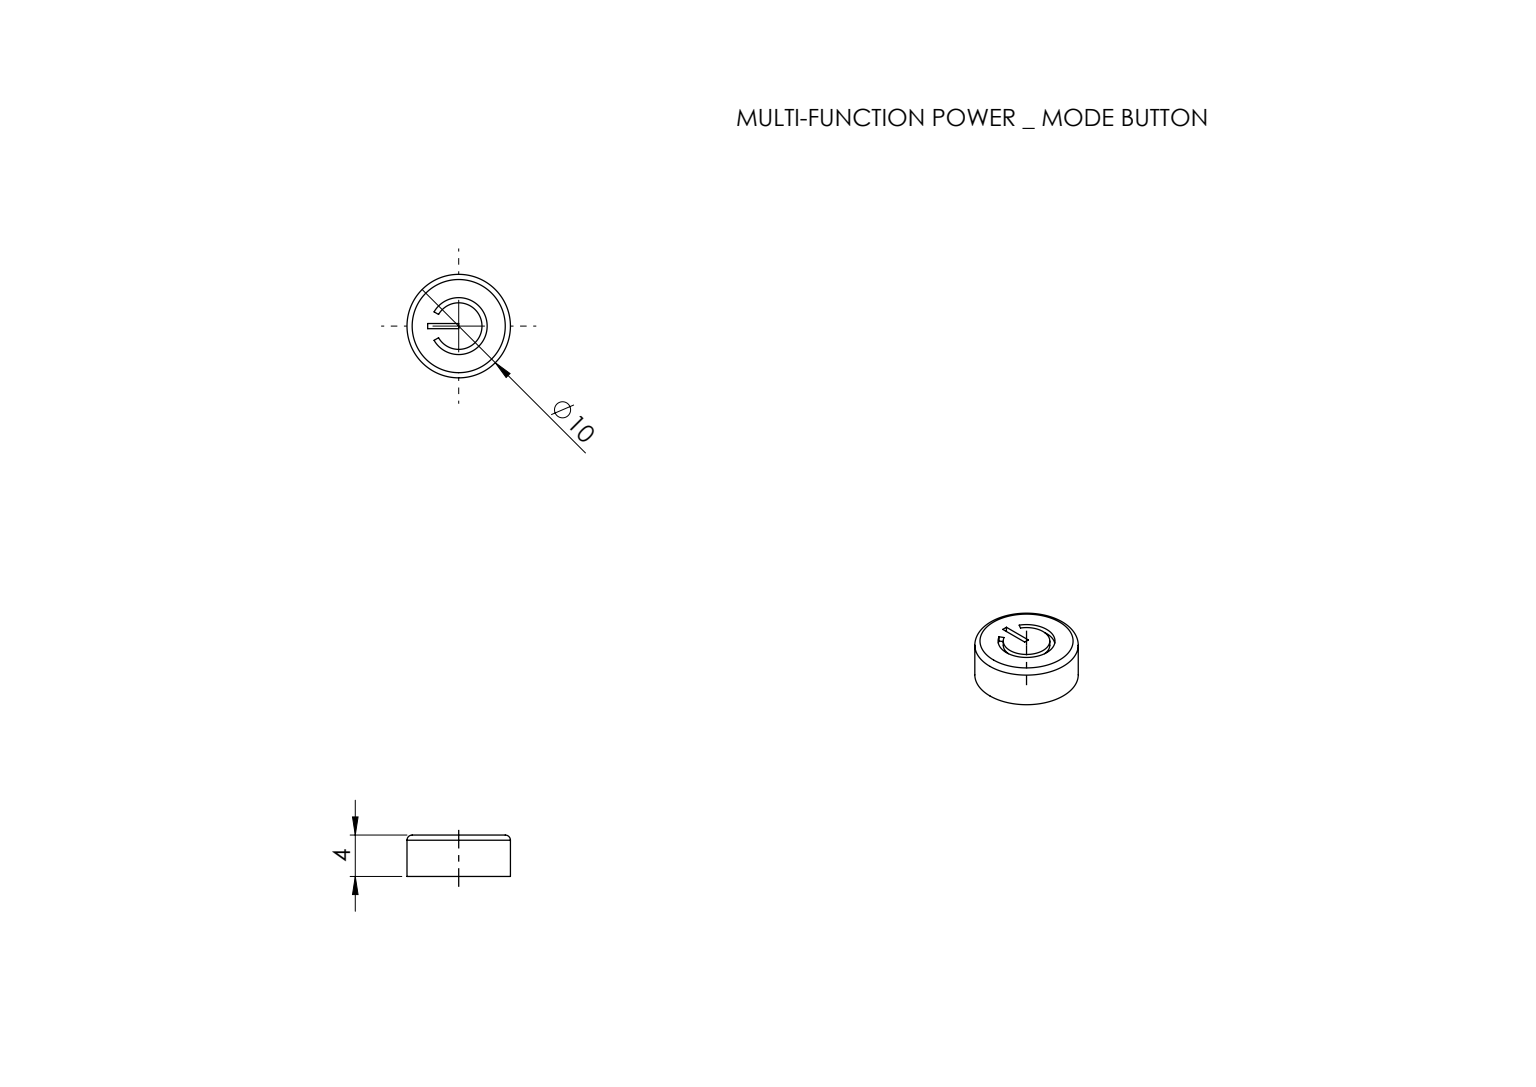
ISO-10303-21;
HEADER;
FILE_DESCRIPTION (('STEP AP214'),
    '1' );
FILE_NAME ('Multi-Function Power _ Mode Button.step',
    '2026-10-02T09:26:43',
    ( '' ),
    ( '' ),
    'SwSTEP 2.0',
    'SolidWorks 2026',
    '' );
FILE_SCHEMA (( 'AUTOMOTIVE_DESIGN' ));
ENDSEC;

DATA;
#385=ORIENTED_EDGE ( 'NONE', *, *, #77434, .T. ) ;
#488=DIRECTION ( 'NONE',  ( 1.000000000000000000, 0.000000000000000000, 0.000000000000000000 ) ) ;
#790=DIRECTION ( 'NONE',  ( -0.000000000000000000, -1.000000000000000000, -0.000000000000000000 ) ) ;
#881=DIRECTION ( 'NONE',  ( -0.000000000000000000, -1.000000000000000000, -0.000000000000000000 ) ) ;
#1377=EDGE_CURVE ( 'NONE', #21459, #55389, #67444, .T. ) ;
#1508=( NAMED_UNIT ( * ) SI_UNIT ( $, .STERADIAN. ) SOLID_ANGLE_UNIT ( ) );
#1978=( LENGTH_UNIT ( ) NAMED_UNIT ( * ) SI_UNIT ( .MILLI., .METRE. ) );
#2148=VERTEX_POINT ( 'NONE', #84417 ) ;
#2193=DIRECTION ( 'NONE',  ( -0.000000000000000000, -1.000000000000000000, -0.000000000000000000 ) ) ;
#2267=VERTEX_POINT ( 'NONE', #109201 ) ;
#2382=DIRECTION ( 'NONE',  ( 0.000000000000000000, 0.000000000000000000, 1.000000000000000000 ) ) ;
#2384=UNCERTAINTY_MEASURE_WITH_UNIT (LENGTH_MEASURE( 1.000000000000000082E-05 ), #1978, 'distance_accuracy_value', 'NONE');
#2834=APPLICATION_CONTEXT ( 'automotive_design' ) ;
#3149=ORIENTED_EDGE ( 'NONE', *, *, #1377, .F. ) ;
#3203=DIRECTION ( 'NONE',  ( -1.000000000000000000, 0.000000000000000000, 1.224646799147352221E-16 ) ) ;
#3290=DIRECTION ( 'NONE',  ( -0.000000000000000000, -1.000000000000000000, -0.000000000000000000 ) ) ;
#3313=ORIENTED_EDGE ( 'NONE', *, *, #12967, .T. ) ;
#3340=ORIENTED_EDGE ( 'NONE', *, *, #86447, .T. ) ;
#3667=CARTESIAN_POINT ( 'NONE',  ( 105.6184301395928031, 8.500000000000000000, -1.375000000000000888 ) ) ;
#3718=ORIENTED_EDGE ( 'NONE', *, *, #81749, .T. ) ;
#3750=CARTESIAN_POINT ( 'NONE',  ( 106.0514428414850272, 8.500000000000000000, -1.125000000000000222 ) ) ;
#3830=DIRECTION ( 'NONE',  ( -1.224646799147352221E-16, 0.000000000000000000, -1.000000000000000000 ) ) ;
#3880=CIRCLE ( 'NONE', #6023, 0.5000000000000004441 ) ;
#4515=LINE ( 'NONE', #115118, #126781 ) ;
#4690=DIRECTION ( 'NONE',  ( -0.000000000000000000, 1.000000000000000000, -0.000000000000000000 ) ) ;
#4889=EDGE_CURVE ( 'NONE', #106872, #121536, #118797, .T. ) ;
#4891=AXIS2_PLACEMENT_3D ( 'NONE', #71967, #92220, #82437 ) ;
#5329=CARTESIAN_POINT ( 'NONE',  ( 108.0000000000000142, 8.500000000000000000, 0.000000000000000000 ) ) ;
#5405=CARTESIAN_POINT ( 'NONE',  ( 105.0000000000000142, 8.500000000000000000, -0.2499999999999996392 ) ) ;
#5772=CARTESIAN_POINT ( 'NONE',  ( 108.0000000000000142, 5.000000000000000000, 0.000000000000000000 ) ) ;
#5797=EDGE_LOOP ( 'NONE', ( #22080, #113484 ) ) ;
#5964=DIRECTION ( 'NONE',  ( -0.000000000000000000, -1.000000000000000000, -0.000000000000000000 ) ) ;
#5971=( GEOMETRIC_REPRESENTATION_CONTEXT ( 3 ) GLOBAL_UNCERTAINTY_ASSIGNED_CONTEXT ( ( #2384 ) ) GLOBAL_UNIT_ASSIGNED_CONTEXT ( ( #1978, #22299, #60295 ) ) REPRESENTATION_CONTEXT ( 'NONE', 'WORKASPACE' ) );
#5975=FACE_OUTER_BOUND ( 'NONE', #11208, .T. ) ;
#6023=AXIS2_PLACEMENT_3D ( 'NONE', #88627, #38920, #50635 ) ;
#6047=UNCERTAINTY_MEASURE_WITH_UNIT (LENGTH_MEASURE( 1.000000000000000082E-05 ), #11976, 'distance_accuracy_value', 'NONE');
#6325=ORIENTED_EDGE ( 'NONE', *, *, #106005, .T. ) ;
#8150=EDGE_CURVE ( 'NONE', #2148, #54782, #127046, .T. ) ;
#8522=EDGE_CURVE ( 'NONE', #106872, #41830, #78934, .T. ) ;
#8952=ORIENTED_EDGE ( 'NONE', *, *, #89643, .T. ) ;
#8954=AXIS2_PLACEMENT_3D ( 'NONE', #36524, #76432, #77074 ) ;
#9891=ORIENTED_EDGE ( 'NONE', *, *, #89462, .T. ) ;
#10025=VERTEX_POINT ( 'NONE', #92625 ) ;
#10069=DIRECTION ( 'NONE',  ( 0.000000000000000000, -0.000000000000000000, 1.000000000000000000 ) ) ;
#10097=CARTESIAN_POINT ( 'NONE',  ( 108.0000000000000142, 8.500000000000000000, 0.000000000000000000 ) ) ;
#10308=VERTEX_POINT ( 'NONE', #14043 ) ;
#10568=EDGE_CURVE ( 'NONE', #72837, #121539, #100366, .T. ) ;
#10644=CARTESIAN_POINT ( 'NONE',  ( 0.000000000000000000, 0.000000000000000000, 0.000000000000000000 ) ) ;
#10960=ORIENTED_EDGE ( 'NONE', *, *, #81749, .F. ) ;
#11208=EDGE_LOOP ( 'NONE', ( #44989, #6325, #121739, #15666 ) ) ;
#11396=ORIENTED_EDGE ( 'NONE', *, *, #79481, .F. ) ;
#11481=CARTESIAN_POINT ( 'NONE',  ( 108.0000000000000142, 9.000000000000001776, 4.500000000000003553 ) ) ;
#11637=DIRECTION ( 'NONE',  ( 0.000000000000000000, 1.000000000000000000, 0.000000000000000000 ) ) ;
#11693=CYLINDRICAL_SURFACE ( 'NONE', #74639, 2.749999999999997335 ) ;
#11728=ADVANCED_FACE ( 'NONE', ( #29081, #57229, #39562 ), #19222, .T. ) ;
#11976=( LENGTH_UNIT ( ) NAMED_UNIT ( * ) SI_UNIT ( .MILLI., .METRE. ) );
#12204=CARTESIAN_POINT ( 'NONE',  ( 108.0000000000000142, 9.000000000000001776, 5.000000000000004441 ) ) ;
#12216=CARTESIAN_POINT ( 'NONE',  ( 108.0000000000000142, 5.000000000000000000, 0.000000000000000000 ) ) ;
#12407=CARTESIAN_POINT ( 'NONE',  ( 108.0000000000000142, 8.500000000000000000, 2.249999999999996891 ) ) ;
#12614=PRESENTATION_STYLE_ASSIGNMENT (( #61086 ) ) ;
#12967=EDGE_CURVE ( 'NONE', #112645, #70298, #25079, .T. ) ;
#12984=DIRECTION ( 'NONE',  ( 0.000000000000000000, 0.000000000000000000, 1.000000000000000000 ) ) ;
#13074=( NAMED_UNIT ( * ) PLANE_ANGLE_UNIT ( ) SI_UNIT ( $, .RADIAN. ) );
#13182=DIRECTION ( 'NONE',  ( 0.000000000000000000, 0.000000000000000000, 1.000000000000000000 ) ) ;
#13266=ORIENTED_EDGE ( 'NONE', *, *, #55211, .T. ) ;
#13423=ORIENTED_EDGE ( 'NONE', *, *, #70420, .F. ) ;
#13659=DIRECTION ( 'NONE',  ( 0.4999999999999992228, 0.000000000000000000, -0.8660254037844391517 ) ) ;
#13797=DIRECTION ( 'NONE',  ( -0.000000000000000000, 1.000000000000000000, -0.000000000000000000 ) ) ;
#13876=DIRECTION ( 'NONE',  ( -0.000000000000000000, -1.000000000000000000, -0.000000000000000000 ) ) ;
#14043=CARTESIAN_POINT ( 'NONE',  ( 106.0514428414850272, 9.000000000000001776, 1.124999999999998002 ) ) ;
#15131=DIRECTION ( 'NONE',  ( 1.000000000000000000, 0.000000000000000000, -1.776356839400246520E-15 ) ) ;
#15253=ORIENTED_EDGE ( 'NONE', *, *, #113422, .F. ) ;
#15666=ORIENTED_EDGE ( 'NONE', *, *, #93447, .F. ) ;
#16016=CARTESIAN_POINT ( 'NONE',  ( 105.6184301395928031, 9.000000000000001776, 1.375000000000001110 ) ) ;
#16189=APPLICATION_CONTEXT ( 'automotive_design' ) ;
#16276=ADVANCED_FACE ( 'NONE', ( #21523 ), #11693, .F. ) ;
#16605=EDGE_CURVE ( 'NONE', #74101, #10308, #73370, .T. ) ;
#16684=VECTOR ( 'NONE', #13797, 1000.000000000000000 ) ;
#17289=DIRECTION ( 'NONE',  ( 0.8660254037844390407, 0.000000000000000000, -0.4999999999999991673 ) ) ;
#17307=CIRCLE ( 'NONE', #46578, 5.000000000000004441 ) ;
#17535=FACE_OUTER_BOUND ( 'NONE', #5797, .T. ) ;
#17646=AXIS2_PLACEMENT_3D ( 'NONE', #126359, #117804, #56948 ) ;
#17782=EDGE_LOOP ( 'NONE', ( #128177, #26734, #108737, #88245 ) ) ;
#17911=DIRECTION ( 'NONE',  ( 1.000000000000000000, 0.000000000000000000, 8.881784197001235560E-16 ) ) ;
#18235=LINE ( 'NONE', #70561, #41090 ) ;
#18489=ADVANCED_FACE ( 'NONE', ( #17535 ), #75813, .F. ) ;
#18780=CARTESIAN_POINT ( 'NONE',  ( 105.0000000000000142, 9.000000000000001776, 0.2500000000000003886 ) ) ;
#19087=CARTESIAN_POINT ( 'NONE',  ( 108.0000000000000142, 8.500000000000000000, 0.000000000000000000 ) ) ;
#19205=DIRECTION ( 'NONE',  ( -1.000000000000000000, 0.000000000000000000, 1.224646799147352221E-16 ) ) ;
#19222=PLANE ( 'NONE',  #63419 ) ;
#19401=AXIS2_PLACEMENT_3D ( 'NONE', #5772, #126869, #26096 ) ;
#19403=ORIENTED_EDGE ( 'NONE', *, *, #117219, .T. ) ;
#19505=EDGE_LOOP ( 'NONE', ( #103192, #97868, #89992, #40928 ) ) ;
#19520=DIRECTION ( 'NONE',  ( 0.000000000000000000, 0.000000000000000000, 1.000000000000000000 ) ) ;
#19573=AXIS2_PLACEMENT_3D ( 'NONE', #91743, #83223, #102836 ) ;
#19603=CARTESIAN_POINT ( 'NONE',  ( 108.0000000000000142, 9.000000000000001776, -5.000000000000004441 ) ) ;
#19610=DIRECTION ( 'NONE',  ( -0.000000000000000000, 1.000000000000000000, -0.000000000000000000 ) ) ;
#20007=DIRECTION ( 'NONE',  ( -1.000000000000000000, 0.000000000000000000, 1.224646799147352221E-16 ) ) ;
#20093=LINE ( 'NONE', #89473, #27972 ) ;
#20109=DIRECTION ( 'NONE',  ( -0.000000000000000000, -1.000000000000000000, -0.000000000000000000 ) ) ;
#21087=VECTOR ( 'NONE', #20109, 1000.000000000000000 ) ;
#21272=PRODUCT_DEFINITION_FORMATION_WITH_SPECIFIED_SOURCE ( 'ANY', '', #72268, .NOT_KNOWN. ) ;
#21349=DIRECTION ( 'NONE',  ( 1.000000000000000000, 0.000000000000000000, 8.881784197001235560E-16 ) ) ;
#21459=VERTEX_POINT ( 'NONE', #91482 ) ;
#21523=FACE_OUTER_BOUND ( 'NONE', #121290, .T. ) ;
#21874=VERTEX_POINT ( 'NONE', #11481 ) ;
#22080=ORIENTED_EDGE ( 'NONE', *, *, #114243, .F. ) ;
#22299=( NAMED_UNIT ( * ) PLANE_ANGLE_UNIT ( ) SI_UNIT ( $, .RADIAN. ) );
#22796=VECTOR ( 'NONE', #17289, 1000.000000000000227 ) ;
#22913=LINE ( 'NONE', #62831, #59996 ) ;
#23418=CIRCLE ( 'NONE', #48569, 2.750000000000002665 ) ;
#23447=DIRECTION ( 'NONE',  ( -0.000000000000000000, 1.000000000000000000, -0.000000000000000000 ) ) ;
#23521=CARTESIAN_POINT ( 'NONE',  ( 106.0514428414850272, 8.500000000000000000, 1.125000000000000444 ) ) ;
#23569=CARTESIAN_POINT ( 'NONE',  ( 108.0000000000000142, 9.000000000000001776, 0.000000000000000000 ) ) ;
#24135=DIRECTION ( 'NONE',  ( 0.000000000000000000, 0.000000000000000000, 1.000000000000000000 ) ) ;
#24517=CIRCLE ( 'NONE', #106077, 2.250000000000001776 ) ;
#24540=ORIENTED_EDGE ( 'NONE', *, *, #98030, .T. ) ;
#24891=CARTESIAN_POINT ( 'NONE',  ( 108.0000000000000142, 9.000000000000001776, -0.2500000000000000000 ) ) ;
#24976=EDGE_LOOP ( 'NONE', ( #85852, #95541, #46748, #54051, #3149, #85174, #50534, #49698 ) ) ;
#25079=LINE ( 'NONE', #114103, #116619 ) ;
#25272=DIRECTION ( 'NONE',  ( -0.000000000000000000, -1.000000000000000000, -0.000000000000000000 ) ) ;
#25381=ORIENTED_EDGE ( 'NONE', *, *, #48110, .T. ) ;
#25558=ORIENTED_EDGE ( 'NONE', *, *, #55661, .F. ) ;
#25818=ORIENTED_EDGE ( 'NONE', *, *, #48110, .F. ) ;
#25918=CARTESIAN_POINT ( 'NONE',  ( 108.0000000000000142, 8.500000000000000000, 0.000000000000000000 ) ) ;
#26066=CARTESIAN_POINT ( 'NONE',  ( 108.0000000000000142, 9.000000000000001776, -0.2500000000000000000 ) ) ;
#26096=DIRECTION ( 'NONE',  ( 0.000000000000000000, -0.000000000000000000, 1.000000000000000000 ) ) ;
#26734=ORIENTED_EDGE ( 'NONE', *, *, #117792, .F. ) ;
#26804=EDGE_CURVE ( 'NONE', #109687, #10308, #34412, .T. ) ;
#26823=ORIENTED_EDGE ( 'NONE', *, *, #33540, .F. ) ;
#27919=DIRECTION ( 'NONE',  ( 1.000000000000000000, 0.000000000000000000, 1.776356839400247112E-15 ) ) ;
#27972=VECTOR ( 'NONE', #61953, 1000.000000000000000 ) ;
#28111=ORIENTED_EDGE ( 'NONE', *, *, #83838, .T. ) ;
#28210=EDGE_LOOP ( 'NONE', ( #77891, #123182, #92206, #99342 ) ) ;
#29081=FACE_BOUND ( 'NONE', #88903, .T. ) ;
#29085=EDGE_CURVE ( 'NONE', #55389, #74101, #108331, .T. ) ;
#30179=SHAPE_REPRESENTATION_RELATIONSHIP ( 'NONE' , 'NONE' ,  #89551, #108597 ) ;
#30252=DIRECTION ( 'NONE',  ( 1.000000000000000000, 0.000000000000000000, 0.000000000000000000 ) ) ;
#30311=ORIENTED_EDGE ( 'NONE', *, *, #113227, .T. ) ;
#30359=LINE ( 'NONE', #101005, #116796 ) ;
#30746=CIRCLE ( 'NONE', #124816, 4.500000000000003553 ) ;
#30906=DIRECTION ( 'NONE',  ( -1.000000000000000000, 0.000000000000000000, 0.000000000000000000 ) ) ;
#31194=CARTESIAN_POINT ( 'NONE',  ( 108.0000000000000142, 9.000000000000001776, 0.000000000000000000 ) ) ;
#31397=FACE_OUTER_BOUND ( 'NONE', #28210, .T. ) ;
#31472=CARTESIAN_POINT ( 'NONE',  ( 108.0000000000000142, 9.000000000000001776, -0.2500000000000000000 ) ) ;
#31821=CARTESIAN_POINT ( 'NONE',  ( 105.0000000000000142, 8.500000000000000000, 0.2500000000000003886 ) ) ;
#32513=DIRECTION ( 'NONE',  ( -0.000000000000000000, 1.000000000000000000, -0.000000000000000000 ) ) ;
#33199=STYLED_ITEM ( 'NONE', ( #70731 ), #108597 ) ;
#33298=ORIENTED_EDGE ( 'NONE', *, *, #4889, .F. ) ;
#33482=AXIS2_PLACEMENT_3D ( 'NONE', #47716, #69261, #120319 ) ;
#33540=EDGE_CURVE ( 'NONE', #55389, #56667, #109269, .T. ) ;
#33800=DIRECTION ( 'NONE',  ( 0.000000000000000000, 1.000000000000000000, 0.000000000000000000 ) ) ;
#34131=ORIENTED_EDGE ( 'NONE', *, *, #114243, .T. ) ;
#34206=ORIENTED_EDGE ( 'NONE', *, *, #117219, .F. ) ;
#34412=CIRCLE ( 'NONE', #122223, 2.250000000000001776 ) ;
#34634=ORIENTED_EDGE ( 'NONE', *, *, #12967, .F. ) ;
#34781=ADVANCED_FACE ( 'NONE', ( #31397 ), #61505, .T. ) ;
#34787=ADVANCED_FACE ( 'NONE', ( #113814 ), #94164, .T. ) ;
#34828=DIRECTION ( 'NONE',  ( 1.000000000000000000, 0.000000000000000000, -8.881784197001232602E-16 ) ) ;
#34919=VECTOR ( 'NONE', #67830, 1000.000000000000227 ) ;
#35042=AXIS2_PLACEMENT_3D ( 'NONE', #10097, #110231, #48095 ) ;
#35244=CARTESIAN_POINT ( 'NONE',  ( 108.0000000000000142, 8.500000000000000000, 0.000000000000000000 ) ) ;
#35998=VECTOR ( 'NONE', #104719, 1000.000000000000000 ) ;
#36343=CARTESIAN_POINT ( 'NONE',  ( 105.0000000000000142, 8.500000000000000000, 0.2500000000000003886 ) ) ;
#36524=CARTESIAN_POINT ( 'NONE',  ( 108.0000000000000142, 8.500000000000000000, -0.2500000000000000000 ) ) ;
#37026=DIRECTION ( 'NONE',  ( -0.000000000000000000, 1.000000000000000000, -0.000000000000000000 ) ) ;
#37092=AXIS2_PLACEMENT_3D ( 'NONE', #49730, #83052, #12984 ) ;
#37163=PLANE ( 'NONE',  #8954 ) ;
#37321=AXIS2_PLACEMENT_3D ( 'NONE', #5329, #5964, #15131 ) ;
#37329=AXIS2_PLACEMENT_3D ( 'NONE', #73402, #102854, #13182 ) ;
#37832=ORIENTED_EDGE ( 'NONE', *, *, #102627, .F. ) ;
#38166=VECTOR ( 'NONE', #102869, 1000.000000000000000 ) ;
#38625=CARTESIAN_POINT ( 'NONE',  ( 108.0000000000000142, 9.000000000000001776, -2.749999999999997335 ) ) ;
#38888=DIRECTION ( 'NONE',  ( -0.000000000000000000, -1.000000000000000000, -0.000000000000000000 ) ) ;
#38920=DIRECTION ( 'NONE',  ( 1.000000000000000000, -0.000000000000000000, 1.224646799147353207E-16 ) ) ;
#39345=ORIENTED_EDGE ( 'NONE', *, *, #58572, .T. ) ;
#39562=FACE_OUTER_BOUND ( 'NONE', #40627, .T. ) ;
#39567=ORIENTED_EDGE ( 'NONE', *, *, #58572, .F. ) ;
#40182=CARTESIAN_POINT ( 'NONE',  ( 108.0000000000000142, 9.000000000000001776, 0.000000000000000000 ) ) ;
#40340=ORIENTED_EDGE ( 'NONE', *, *, #84111, .F. ) ;
#40627=EDGE_LOOP ( 'NONE', ( #65864, #59906 ) ) ;
#40750=CARTESIAN_POINT ( 'NONE',  ( 108.0000000000000142, 8.500000000000000000, 0.000000000000000000 ) ) ;
#40928=ORIENTED_EDGE ( 'NONE', *, *, #83838, .F. ) ;
#41090=VECTOR ( 'NONE', #98089, 1000.000000000000000 ) ;
#41376=FACE_OUTER_BOUND ( 'NONE', #110535, .T. ) ;
#41470=FILL_AREA_STYLE ('',( #62387 ) ) ;
#41524=COLOUR_RGB ( '', 0.09019608, 0.27058824, 0.51372549) ;
#41633=ORIENTED_EDGE ( 'NONE', *, *, #63862, .T. ) ;
#41830=VERTEX_POINT ( 'NONE', #89807 ) ;
#41929=SURFACE_SIDE_STYLE ('',( #120477 ) ) ;
#42228=EDGE_LOOP ( 'NONE', ( #127274, #26823, #98448, #63687 ) ) ;
#43209=DIRECTION ( 'NONE',  ( -0.000000000000000000, 1.000000000000000000, -0.000000000000000000 ) ) ;
#43297=DIRECTION ( 'NONE',  ( 1.000000000000000000, 0.000000000000000000, 0.000000000000000000 ) ) ;
#43711=DIRECTION ( 'NONE',  ( 0.4999999999999992228, 0.000000000000000000, 0.8660254037844391517 ) ) ;
#43962=FACE_OUTER_BOUND ( 'NONE', #89837, .T. ) ;
#44989=ORIENTED_EDGE ( 'NONE', *, *, #79481, .T. ) ;
#45073=LINE ( 'NONE', #26066, #120884 ) ;
#45696=VERTEX_POINT ( 'NONE', #87212 ) ;
#45888=CARTESIAN_POINT ( 'NONE',  ( 105.0000000000000142, 9.000000000000001776, -0.2499999999999996392 ) ) ;
#45948=DIRECTION ( 'NONE',  ( 0.000000000000000000, 0.000000000000000000, 1.000000000000000000 ) ) ;
#46326=ORIENTED_EDGE ( 'NONE', *, *, #61733, .F. ) ;
#46442=EDGE_LOOP ( 'NONE', ( #37832, #34206, #83731, #75654 ) ) ;
#46490=CIRCLE ( 'NONE', #73584, 2.750000000000002665 ) ;
#46549=DIRECTION ( 'NONE',  ( 0.000000000000000000, 0.000000000000000000, -1.000000000000000000 ) ) ;
#46578=AXIS2_PLACEMENT_3D ( 'NONE', #60272, #100790, #78616 ) ;
#46623=ORIENTED_EDGE ( 'NONE', *, *, #106834, .T. ) ;
#46748=ORIENTED_EDGE ( 'NONE', *, *, #61733, .T. ) ;
#47511=CARTESIAN_POINT ( 'NONE',  ( 108.0000000000000142, 8.500000000000000000, 0.2500000000000000000 ) ) ;
#47716=CARTESIAN_POINT ( 'NONE',  ( 108.0000000000000142, 5.000000000000000000, 0.000000000000000000 ) ) ;
#48095=DIRECTION ( 'NONE',  ( 0.000000000000000000, 0.000000000000000000, 1.000000000000000000 ) ) ;
#48110=EDGE_CURVE ( 'NONE', #45696, #10025, #110733, .T. ) ;
#48569=AXIS2_PLACEMENT_3D ( 'NONE', #40750, #790, #81924 ) ;
#48733=VECTOR ( 'NONE', #59560, 1000.000000000000000 ) ;
#48807=ADVANCED_FACE ( 'NONE', ( #43962 ), #101588, .F. ) ;
#48855=LINE ( 'NONE', #80241, #34919 ) ;
#49540=PLANE ( 'NONE',  #106935 ) ;
#49630=CIRCLE ( 'NONE', #66326, 2.750000000000002665 ) ;
#49698=ORIENTED_EDGE ( 'NONE', *, *, #89643, .F. ) ;
#49730=CARTESIAN_POINT ( 'NONE',  ( 108.0000000000000142, 9.000000000000001776, 0.000000000000000000 ) ) ;
#49771=COLOUR_RGB ( '', 0.09019608, 0.27058824, 0.51372549) ;
#49971=EDGE_LOOP ( 'NONE', ( #64267, #13266, #30311, #78729 ) ) ;
#50264=CARTESIAN_POINT ( 'NONE',  ( 108.0000000000000142, 8.500000000000000000, -2.249999999999996891 ) ) ;
#50333=EDGE_CURVE ( 'NONE', #84351, #2148, #95891, .T. ) ;
#50498=VERTEX_POINT ( 'NONE', #81512 ) ;
#50534=ORIENTED_EDGE ( 'NONE', *, *, #106834, .F. ) ;
#50635=DIRECTION ( 'NONE',  ( 0.000000000000000000, 0.000000000000000000, -1.000000000000000000 ) ) ;
#51125=CARTESIAN_POINT ( 'NONE',  ( 105.0000000000000142, 8.500000000000000000, 0.2500000000000003886 ) ) ;
#51191=VECTOR ( 'NONE', #37026, 1000.000000000000000 ) ;
#51210=EDGE_CURVE ( 'NONE', #2267, #121831, #77284, .T. ) ;
#51471=ADVANCED_FACE ( 'NONE', ( #63323 ), #83622, .T. ) ;
#51679=CARTESIAN_POINT ( 'NONE',  ( 106.0514428414850272, 8.500000000000000000, -1.125000000000000222 ) ) ;
#51940=AXIS2_PLACEMENT_3D ( 'NONE', #23569, #3290, #73304 ) ;
#52200=ADVANCED_FACE ( 'NONE', ( #56558 ), #87310, .F. ) ;
#52335=AXIS2_PLACEMENT_3D ( 'NONE', #82979, #43711, #81670 ) ;
#52617=VECTOR ( 'NONE', #20007, 1000.000000000000000 ) ;
#52694=ORIENTED_EDGE ( 'NONE', *, *, #77434, .F. ) ;
#53039=CYLINDRICAL_SURFACE ( 'NONE', #51940, 5.000000000000004441 ) ;
#54051=ORIENTED_EDGE ( 'NONE', *, *, #29085, .F. ) ;
#54782=VERTEX_POINT ( 'NONE', #12407 ) ;
#54852=DIRECTION ( 'NONE',  ( 0.000000000000000000, 1.000000000000000000, 0.000000000000000000 ) ) ;
#55211=EDGE_CURVE ( 'NONE', #2148, #115931, #62670, .T. ) ;
#55389=VERTEX_POINT ( 'NONE', #124151 ) ;
#55661=EDGE_CURVE ( 'NONE', #76546, #115931, #126416, .T. ) ;
#55852=AXIS2_PLACEMENT_3D ( 'NONE', #92872, #3830, #3203 ) ;
#56374=DIRECTION ( 'NONE',  ( -0.000000000000000000, -1.000000000000000000, -0.000000000000000000 ) ) ;
#56455=ORIENTED_EDGE ( 'NONE', *, *, #26804, .F. ) ;
#56558=FACE_OUTER_BOUND ( 'NONE', #17782, .T. ) ;
#56667=VERTEX_POINT ( 'NONE', #113715 ) ;
#56771=DIRECTION ( 'NONE',  ( 0.000000000000000000, 0.000000000000000000, 1.000000000000000000 ) ) ;
#56948=DIRECTION ( 'NONE',  ( 1.000000000000000000, 0.000000000000000000, 0.000000000000000000 ) ) ;
#57229=FACE_BOUND ( 'NONE', #91684, .T. ) ;
#57343=CARTESIAN_POINT ( 'NONE',  ( 108.0000000000000142, 8.500000000000000000, -0.2500000000000000000 ) ) ;
#57403=FACE_OUTER_BOUND ( 'NONE', #116969, .T. ) ;
#57552=VECTOR ( 'NONE', #74957, 1000.000000000000000 ) ;
#58552=DIRECTION ( 'NONE',  ( -0.8660254037844390407, 0.000000000000000000, -0.4999999999999991673 ) ) ;
#58572=EDGE_CURVE ( 'NONE', #72837, #62517, #102249, .T. ) ;
#58606=CARTESIAN_POINT ( 'NONE',  ( 105.6184301395928031, 8.500000000000000000, 1.375000000000001110 ) ) ;
#58789=AXIS2_PLACEMENT_3D ( 'NONE', #67671, #127262, #77497 ) ;
#59212=ADVANCED_FACE ( 'NONE', ( #41376 ), #75995, .T. ) ;
#59216=DIRECTION ( 'NONE',  ( -1.000000000000000000, 0.000000000000000000, 0.000000000000000000 ) ) ;
#59560=DIRECTION ( 'NONE',  ( -0.000000000000000000, -1.000000000000000000, -0.000000000000000000 ) ) ;
#59873=FACE_OUTER_BOUND ( 'NONE', #84713, .T. ) ;
#59906=ORIENTED_EDGE ( 'NONE', *, *, #70420, .T. ) ;
#59996=VECTOR ( 'NONE', #43209, 1000.000000000000000 ) ;
#60272=CARTESIAN_POINT ( 'NONE',  ( 108.0000000000000142, 8.500000000000000000, 0.000000000000000000 ) ) ;
#60295=( NAMED_UNIT ( * ) SI_UNIT ( $, .STERADIAN. ) SOLID_ANGLE_UNIT ( ) );
#60761=AXIS2_PLACEMENT_3D ( 'NONE', #19087, #79344, #30252 ) ;
#60986=DIRECTION ( 'NONE',  ( 0.000000000000000000, 0.000000000000000000, 1.000000000000000000 ) ) ;
#61086=SURFACE_STYLE_USAGE ( .BOTH. , #63018 ) ;
#61261=PRODUCT_DEFINITION ( 'UNKNOWN', '', #21272, #85987 ) ;
#61287=DIRECTION ( 'NONE',  ( 1.000000000000000000, 0.000000000000000000, 0.000000000000000000 ) ) ;
#61505=CYLINDRICAL_SURFACE ( 'NONE', #4891, 2.249999999999996891 ) ;
#61521=AXIS2_PLACEMENT_3D ( 'NONE', #127871, #38888, #17911 ) ;
#61733=EDGE_CURVE ( 'NONE', #54782, #74101, #24517, .T. ) ;
#61792=FACE_OUTER_BOUND ( 'NONE', #19505, .T. ) ;
#61934=FACE_OUTER_BOUND ( 'NONE', #46442, .T. ) ;
#61953=DIRECTION ( 'NONE',  ( 0.000000000000000000, 0.000000000000000000, -1.000000000000000000 ) ) ;
#62021=DIRECTION ( 'NONE',  ( -0.000000000000000000, 1.000000000000000000, -0.000000000000000000 ) ) ;
#62387=FILL_AREA_STYLE_COLOUR ( '', #49771 ) ;
#62517=VERTEX_POINT ( 'NONE', #76020 ) ;
#62651=AXIS2_PLACEMENT_3D ( 'NONE', #105856, #68498, #96654 ) ;
#62670=LINE ( 'NONE', #50264, #92884 ) ;
#62831=CARTESIAN_POINT ( 'NONE',  ( 108.0000000000000142, 8.500000000000000000, 2.249999999999996891 ) ) ;
#63018=SURFACE_SIDE_STYLE ('',( #91190 ) ) ;
#63036=VECTOR ( 'NONE', #19610, 1000.000000000000000 ) ;
#63323=FACE_OUTER_BOUND ( 'NONE', #42228, .T. ) ;
#63419=AXIS2_PLACEMENT_3D ( 'NONE', #40182, #88626, #10069 ) ;
#63645=CARTESIAN_POINT ( 'NONE',  ( 108.0000000000000142, 9.000000000000001776, 0.000000000000000000 ) ) ;
#63687=ORIENTED_EDGE ( 'NONE', *, *, #16605, .T. ) ;
#63700=LINE ( 'NONE', #5405, #105671 ) ;
#63862=EDGE_CURVE ( 'NONE', #62517, #108936, #30359, .T. ) ;
#64110=DIRECTION ( 'NONE',  ( 0.000000000000000000, 0.000000000000000000, 1.000000000000000000 ) ) ;
#64267=ORIENTED_EDGE ( 'NONE', *, *, #8150, .F. ) ;
#64321=MECHANICAL_DESIGN_GEOMETRIC_PRESENTATION_REPRESENTATION('',(#70589),#116544);
#64587=VERTEX_POINT ( 'NONE', #66074 ) ;
#65214=TOROIDAL_SURFACE ( 'NONE', #96604, 4.500000000000003553, 0.5000000000000000000 ) ;
#65531=ORIENTED_EDGE ( 'NONE', *, *, #106005, .F. ) ;
#65712=ORIENTED_EDGE ( 'NONE', *, *, #26804, .T. ) ;
#65864=ORIENTED_EDGE ( 'NONE', *, *, #84111, .T. ) ;
#65966=EDGE_CURVE ( 'NONE', #121536, #107284, #66740, .T. ) ;
#66064=FACE_OUTER_BOUND ( 'NONE', #70387, .T. ) ;
#66074=CARTESIAN_POINT ( 'NONE',  ( 108.0000000000000142, 9.000000000000001776, -4.500000000000003553 ) ) ;
#66326=AXIS2_PLACEMENT_3D ( 'NONE', #31194, #71099, #21349 ) ;
#66412=LINE ( 'NONE', #36343, #57552 ) ;
#66612=CARTESIAN_POINT ( 'NONE',  ( 105.6184301395928031, 9.000000000000001776, -1.375000000000000888 ) ) ;
#66740=LINE ( 'NONE', #24891, #35998 ) ;
#66818=CARTESIAN_POINT ( 'NONE',  ( 108.0000000000000142, 9.000000000000001776, 0.000000000000000000 ) ) ;
#67059=ADVANCED_FACE ( 'NONE', ( #74757 ), #96308, .T. ) ;
#67444=CIRCLE ( 'NONE', #61521, 2.750000000000002665 ) ;
#67671=CARTESIAN_POINT ( 'NONE',  ( 108.0000000000000142, 8.500000000000000000, -0.2500000000000000000 ) ) ;
#67765=DIRECTION ( 'NONE',  ( 0.000000000000000000, 0.000000000000000000, 1.000000000000000000 ) ) ;
#67830=DIRECTION ( 'NONE',  ( -0.8660254037844390407, 0.000000000000000000, -0.4999999999999991673 ) ) ;
#68004=AXIS2_PLACEMENT_3D ( 'NONE', #63645, #13876, #112095 ) ;
#68498=DIRECTION ( 'NONE',  ( -0.000000000000000000, 1.000000000000000000, -0.000000000000000000 ) ) ;
#68669=CLOSED_SHELL ( 'NONE', ( #16276, #48807, #67059, #118857, #59212, #126596, #85161, #11728, #18489, #102884, #52200, #104542, #70470, #107654, #101771, #34781, #34787, #100184, #51471, #113671 ) ) ;
#68700=DIRECTION ( 'NONE',  ( 0.000000000000000000, 0.000000000000000000, -1.000000000000000000 ) ) ;
#68869=DIRECTION ( 'NONE',  ( 1.000000000000000000, 0.000000000000000000, 0.000000000000000000 ) ) ;
#68994=LINE ( 'NONE', #120684, #108539 ) ;
#69096=CARTESIAN_POINT ( 'NONE',  ( 106.0514428414850272, 8.500000000000000000, -1.125000000000000222 ) ) ;
#69261=DIRECTION ( 'NONE',  ( 0.000000000000000000, 1.000000000000000000, 0.000000000000000000 ) ) ;
#69325=LINE ( 'NONE', #19603, #48733 ) ;
#69347=EDGE_CURVE ( 'NONE', #76682, #56667, #49630, .T. ) ;
#70266=( NAMED_UNIT ( * ) PLANE_ANGLE_UNIT ( ) SI_UNIT ( $, .RADIAN. ) );
#70298=VERTEX_POINT ( 'NONE', #38625 ) ;
#70311=CARTESIAN_POINT ( 'NONE',  ( 0.000000000000000000, 8.500000000000000000, 0.000000000000000000 ) ) ;
#70387=EDGE_LOOP ( 'NONE', ( #65531, #25381, #83169, #34131 ) ) ;
#70420=EDGE_CURVE ( 'NONE', #64587, #21874, #83067, .T. ) ;
#70470=ADVANCED_FACE ( 'NONE', ( #103329 ), #124257, .T. ) ;
#70561=CARTESIAN_POINT ( 'NONE',  ( 108.0000000000000142, 8.500000000000000000, 2.749999999999997335 ) ) ;
#70589=STYLED_ITEM ( 'NONE', ( #12614 ), #99052 ) ;
#70731=PRESENTATION_STYLE_ASSIGNMENT (( #100196 ) ) ;
#71099=DIRECTION ( 'NONE',  ( -0.000000000000000000, -1.000000000000000000, -0.000000000000000000 ) ) ;
#71108=EDGE_CURVE ( 'NONE', #121536, #62517, #45073, .T. ) ;
#71472=CIRCLE ( 'NONE', #84086, 5.000000000000004441 ) ;
#71967=CARTESIAN_POINT ( 'NONE',  ( 108.0000000000000142, 8.500000000000000000, 0.000000000000000000 ) ) ;
#72130=ORIENTED_EDGE ( 'NONE', *, *, #98488, .T. ) ;
#72268=PRODUCT ( 'Multi-Function Power _ Mode Button', 'Multi-Function Power _ Mode Button', '', ( #108567 ) ) ;
#72837=VERTEX_POINT ( 'NONE', #47511 ) ;
#73304=DIRECTION ( 'NONE',  ( 0.000000000000000000, 0.000000000000000000, -1.000000000000000000 ) ) ;
#73370=LINE ( 'NONE', #103489, #16684 ) ;
#73402=CARTESIAN_POINT ( 'NONE',  ( 108.0000000000000142, 8.500000000000000000, 0.000000000000000000 ) ) ;
#73521=DIRECTION ( 'NONE',  ( -0.000000000000000000, 1.000000000000000000, -0.000000000000000000 ) ) ;
#73584=AXIS2_PLACEMENT_3D ( 'NONE', #89956, #101076, #43297 ) ;
#74101=VERTEX_POINT ( 'NONE', #23521 ) ;
#74625=EDGE_LOOP ( 'NONE', ( #89203, #76637, #8952, #385 ) ) ;
#74639=AXIS2_PLACEMENT_3D ( 'NONE', #113114, #23447, #123568 ) ;
#74757=FACE_OUTER_BOUND ( 'NONE', #49971, .T. ) ;
#74810=ORIENTED_EDGE ( 'NONE', *, *, #98030, .F. ) ;
#74948=( GEOMETRIC_REPRESENTATION_CONTEXT ( 3 ) GLOBAL_UNCERTAINTY_ASSIGNED_CONTEXT ( ( #82270 ) ) GLOBAL_UNIT_ASSIGNED_CONTEXT ( ( #92961, #13074, #102127 ) ) REPRESENTATION_CONTEXT ( 'NONE', 'WORKASPACE' ) );
#74957=DIRECTION ( 'NONE',  ( -0.000000000000000000, 1.000000000000000000, -0.000000000000000000 ) ) ;
#75654=ORIENTED_EDGE ( 'NONE', *, *, #117792, .T. ) ;
#75813=PLANE ( 'NONE',  #19401 ) ;
#75841=EDGE_LOOP ( 'NONE', ( #78929, #33298, #28111, #39345 ) ) ;
#75995=TOROIDAL_SURFACE ( 'NONE', #19573, 4.500000000000003553, 0.5000000000000000000 ) ;
#76020=CARTESIAN_POINT ( 'NONE',  ( 108.0000000000000142, 9.000000000000001776, 0.2500000000000000000 ) ) ;
#76021=CARTESIAN_POINT ( 'NONE',  ( 108.0000000000000142, 9.000000000000001776, 0.000000000000000000 ) ) ;
#76042=CARTESIAN_POINT ( 'NONE',  ( 108.0000000000000142, 8.500000000000000000, 0.000000000000000000 ) ) ;
#76356=DIRECTION ( 'NONE',  ( -0.000000000000000000, 1.000000000000000000, -0.000000000000000000 ) ) ;
#76401=CYLINDRICAL_SURFACE ( 'NONE', #62651, 2.749999999999997335 ) ;
#76432=DIRECTION ( 'NONE',  ( -1.000000000000000000, 0.000000000000000000, 0.000000000000000000 ) ) ;
#76546=VERTEX_POINT ( 'NONE', #113939 ) ;
#76637=ORIENTED_EDGE ( 'NONE', *, *, #79763, .F. ) ;
#76682=VERTEX_POINT ( 'NONE', #86394 ) ;
#77074=DIRECTION ( 'NONE',  ( 0.000000000000000000, 0.000000000000000000, 1.000000000000000000 ) ) ;
#77284=CIRCLE ( 'NONE', #33482, 5.000000000000004441 ) ;
#77288=AXIS2_PLACEMENT_3D ( 'NONE', #25918, #116854, #67765 ) ;
#77434=EDGE_CURVE ( 'NONE', #50498, #102801, #111695, .T. ) ;
#77497=DIRECTION ( 'NONE',  ( -1.000000000000000000, 0.000000000000000000, 1.224646799147352221E-16 ) ) ;
#77623=LINE ( 'NONE', #69096, #111518 ) ;
#77886=PLANE ( 'NONE',  #17646 ) ;
#77891=ORIENTED_EDGE ( 'NONE', *, *, #55211, .F. ) ;
#77893=EDGE_CURVE ( 'NONE', #70298, #76682, #46490, .T. ) ;
#78616=DIRECTION ( 'NONE',  ( 0.000000000000000000, 0.000000000000000000, 1.000000000000000000 ) ) ;
#78729=ORIENTED_EDGE ( 'NONE', *, *, #83892, .F. ) ;
#78765=EDGE_LOOP ( 'NONE', ( #106510, #39567, #92341, #19403 ) ) ;
#78929=ORIENTED_EDGE ( 'NONE', *, *, #71108, .F. ) ;
#78934=LINE ( 'NONE', #57343, #52617 ) ;
#79344=DIRECTION ( 'NONE',  ( -0.000000000000000000, -1.000000000000000000, -0.000000000000000000 ) ) ;
#79481=EDGE_CURVE ( 'NONE', #10025, #45696, #17307, .T. ) ;
#79763=EDGE_CURVE ( 'NONE', #84351, #76546, #77623, .T. ) ;
#79859=VECTOR ( 'NONE', #90529, 1000.000000000000000 ) ;
#80241=CARTESIAN_POINT ( 'NONE',  ( 106.0514428414850272, 9.000000000000001776, -1.125000000000000222 ) ) ;
#80718=DIRECTION ( 'NONE',  ( 1.000000000000000000, 0.000000000000000000, 0.000000000000000000 ) ) ;
#81512=CARTESIAN_POINT ( 'NONE',  ( 105.6184301395928031, 8.500000000000000000, -1.375000000000000888 ) ) ;
#81557=AXIS2_PLACEMENT_3D ( 'NONE', #120558, #30906, #60986 ) ;
#81663=CARTESIAN_POINT ( 'NONE',  ( 108.0000000000000142, 9.000000000000001776, 0.000000000000000000 ) ) ;
#81670=DIRECTION ( 'NONE',  ( 0.8660254037844391517, 0.000000000000000000, -0.4999999999999992228 ) ) ;
#81749=EDGE_CURVE ( 'NONE', #102801, #70298, #101383, .T. ) ;
#81924=DIRECTION ( 'NONE',  ( 1.000000000000000000, 0.000000000000000000, 1.776356839400247112E-15 ) ) ;
#82270=UNCERTAINTY_MEASURE_WITH_UNIT (LENGTH_MEASURE( 1.000000000000000082E-05 ), #92961, 'distance_accuracy_value', 'NONE');
#82347=AXIS2_PLACEMENT_3D ( 'NONE', #76042, #4690, #45948 ) ;
#82437=DIRECTION ( 'NONE',  ( 0.000000000000000000, 0.000000000000000000, 1.000000000000000000 ) ) ;
#82979=CARTESIAN_POINT ( 'NONE',  ( 105.6184301395928031, 8.500000000000000000, 1.375000000000001110 ) ) ;
#83052=DIRECTION ( 'NONE',  ( 0.000000000000000000, 1.000000000000000000, 0.000000000000000000 ) ) ;
#83067=CIRCLE ( 'NONE', #37092, 4.500000000000003553 ) ;
#83169=ORIENTED_EDGE ( 'NONE', *, *, #93447, .T. ) ;
#83223=DIRECTION ( 'NONE',  ( 0.000000000000000000, 1.000000000000000000, 0.000000000000000000 ) ) ;
#83622=PLANE ( 'NONE',  #52335 ) ;
#83731=ORIENTED_EDGE ( 'NONE', *, *, #93940, .T. ) ;
#83838=EDGE_CURVE ( 'NONE', #106872, #72837, #4515, .T. ) ;
#83889=ORIENTED_EDGE ( 'NONE', *, *, #33540, .T. ) ;
#83892=EDGE_CURVE ( 'NONE', #54782, #109687, #22913, .T. ) ;
#84086=AXIS2_PLACEMENT_3D ( 'NONE', #12216, #33800, #2382 ) ;
#84111=EDGE_CURVE ( 'NONE', #21874, #64587, #30746, .T. ) ;
#84351=VERTEX_POINT ( 'NONE', #3750 ) ;
#84417=CARTESIAN_POINT ( 'NONE',  ( 108.0000000000000142, 8.500000000000000000, -2.249999999999996891 ) ) ;
#84713=EDGE_LOOP ( 'NONE', ( #46326, #88168, #65712, #95405 ) ) ;
#85161=ADVANCED_FACE ( 'NONE', ( #66064 ), #53039, .T. ) ;
#85174=ORIENTED_EDGE ( 'NONE', *, *, #102084, .F. ) ;
#85852=ORIENTED_EDGE ( 'NONE', *, *, #50333, .T. ) ;
#85987=PRODUCT_DEFINITION_CONTEXT ( 'detailed design', #16189, 'design' ) ;
#86120=CARTESIAN_POINT ( 'NONE',  ( 108.0000000000000142, 8.500000000000000000, 0.000000000000000000 ) ) ;
#86349=CARTESIAN_POINT ( 'NONE',  ( 108.0000000000000142, 5.000000000000000000, -5.000000000000004441 ) ) ;
#86394=CARTESIAN_POINT ( 'NONE',  ( 108.0000000000000142, 9.000000000000001776, 2.749999999999997335 ) ) ;
#86447=EDGE_CURVE ( 'NONE', #10025, #64587, #3880, .T. ) ;
#87212=CARTESIAN_POINT ( 'NONE',  ( 108.0000000000000142, 8.500000000000000000, 5.000000000000004441 ) ) ;
#87310=PLANE ( 'NONE',  #58789 ) ;
#87523=FACE_OUTER_BOUND ( 'NONE', #75841, .T. ) ;
#87706=AXIS2_PLACEMENT_3D ( 'NONE', #108787, #106851, #68869 ) ;
#87835=AXIS2_PLACEMENT_3D ( 'NONE', #70311, #2193, #59216 ) ;
#88168=ORIENTED_EDGE ( 'NONE', *, *, #83892, .T. ) ;
#88245=ORIENTED_EDGE ( 'NONE', *, *, #4889, .T. ) ;
#88321=LINE ( 'NONE', #109932, #121561 ) ;
#88626=DIRECTION ( 'NONE',  ( 0.000000000000000000, 1.000000000000000000, 0.000000000000000000 ) ) ;
#88627=CARTESIAN_POINT ( 'NONE',  ( 108.0000000000000142, 8.500000000000000000, -4.500000000000003553 ) ) ;
#88889=DIRECTION ( 'NONE',  ( -0.000000000000000000, -1.000000000000000000, -0.000000000000000000 ) ) ;
#88903=EDGE_LOOP ( 'NONE', ( #25558, #72130, #3718, #108996, #122837, #9891, #56455, #124091 ) ) ;
#89203=ORIENTED_EDGE ( 'NONE', *, *, #98488, .F. ) ;
#89462=EDGE_CURVE ( 'NONE', #56667, #10308, #117421, .T. ) ;
#89473=CARTESIAN_POINT ( 'NONE',  ( 105.0000000000000142, 8.500000000000000000, 0.2500000000000003886 ) ) ;
#89551=SHAPE_REPRESENTATION ( 'Multi-Function Power _ Mode Button', ( #108296 ), #5971 ) ;
#89643=EDGE_CURVE ( 'NONE', #84351, #50498, #68994, .T. ) ;
#89807=CARTESIAN_POINT ( 'NONE',  ( 105.0000000000000142, 8.500000000000000000, -0.2499999999999996392 ) ) ;
#89837=EDGE_LOOP ( 'NONE', ( #34634, #92974, #24540, #118389 ) ) ;
#89887=CARTESIAN_POINT ( 'NONE',  ( 108.0000000000000142, 8.500000000000000000, 0.2500000000000000000 ) ) ;
#89956=CARTESIAN_POINT ( 'NONE',  ( 108.0000000000000142, 9.000000000000001776, 0.000000000000000000 ) ) ;
#89992=ORIENTED_EDGE ( 'NONE', *, *, #10568, .F. ) ;
#90152=CARTESIAN_POINT ( 'NONE',  ( 108.0000000000000142, 8.500000000000000000, 0.000000000000000000 ) ) ;
#90516=DIRECTION ( 'NONE',  ( 0.000000000000000000, 0.000000000000000000, 1.000000000000000000 ) ) ;
#90529=DIRECTION ( 'NONE',  ( -1.000000000000000000, 0.000000000000000000, 1.224646799147352221E-16 ) ) ;
#91190=SURFACE_STYLE_FILL_AREA ( #41470 ) ;
#91482=CARTESIAN_POINT ( 'NONE',  ( 108.0000000000000142, 8.500000000000000000, 2.749999999999997335 ) ) ;
#91657=FILL_AREA_STYLE ('',( #100816 ) ) ;
#91684=EDGE_LOOP ( 'NONE', ( #93010, #128617, #41633, #115553 ) ) ;
#91743=CARTESIAN_POINT ( 'NONE',  ( 108.0000000000000142, 8.500000000000000000, 0.000000000000000000 ) ) ;
#91774=CARTESIAN_POINT ( 'NONE',  ( 108.0000000000000142, 8.500000000000000000, 0.2500000000000000000 ) ) ;
#92206=ORIENTED_EDGE ( 'NONE', *, *, #79763, .T. ) ;
#92220=DIRECTION ( 'NONE',  ( -0.000000000000000000, 1.000000000000000000, -0.000000000000000000 ) ) ;
#92341=ORIENTED_EDGE ( 'NONE', *, *, #10568, .T. ) ;
#92625=CARTESIAN_POINT ( 'NONE',  ( 108.0000000000000142, 8.500000000000000000, -5.000000000000004441 ) ) ;
#92745=ORIENTED_EDGE ( 'NONE', *, *, #113422, .T. ) ;
#92872=CARTESIAN_POINT ( 'NONE',  ( 108.0000000000000142, 8.500000000000000000, 0.2500000000000000000 ) ) ;
#92884=VECTOR ( 'NONE', #62021, 1000.000000000000000 ) ;
#92961=( LENGTH_UNIT ( ) NAMED_UNIT ( * ) SI_UNIT ( .MILLI., .METRE. ) );
#92974=ORIENTED_EDGE ( 'NONE', *, *, #102084, .T. ) ;
#93010=ORIENTED_EDGE ( 'NONE', *, *, #65966, .F. ) ;
#93447=EDGE_CURVE ( 'NONE', #10025, #121831, #69325, .T. ) ;
#93589=AXIS2_PLACEMENT_3D ( 'NONE', #90152, #88889, #488 ) ;
#93940=EDGE_CURVE ( 'NONE', #121539, #41830, #20093, .T. ) ;
#93979=CIRCLE ( 'NONE', #87706, 2.250000000000001776 ) ;
#94164=PLANE ( 'NONE',  #121989 ) ;
#94356=DIRECTION ( 'NONE',  ( -0.000000000000000000, -1.000000000000000000, -0.000000000000000000 ) ) ;
#95118=CARTESIAN_POINT ( 'NONE',  ( 108.0000000000000142, 9.000000000000001776, 2.249999999999996891 ) ) ;
#95405=ORIENTED_EDGE ( 'NONE', *, *, #16605, .F. ) ;
#95541=ORIENTED_EDGE ( 'NONE', *, *, #8150, .T. ) ;
#95666=CYLINDRICAL_SURFACE ( 'NONE', #127982, 5.000000000000004441 ) ;
#95891=CIRCLE ( 'NONE', #37321, 2.250000000000001776 ) ;
#96308=CYLINDRICAL_SURFACE ( 'NONE', #82347, 2.249999999999996891 ) ;
#96471=VECTOR ( 'NONE', #32513, 1000.000000000000000 ) ;
#96604=AXIS2_PLACEMENT_3D ( 'NONE', #35244, #54852, #56771 ) ;
#96654=DIRECTION ( 'NONE',  ( 0.000000000000000000, 0.000000000000000000, 1.000000000000000000 ) ) ;
#97200=PRODUCT_DEFINITION_SHAPE ( 'NONE', 'NONE',  #61261 ) ;
#97367=FACE_OUTER_BOUND ( 'NONE', #98862, .T. ) ;
#97868=ORIENTED_EDGE ( 'NONE', *, *, #93940, .F. ) ;
#98030=EDGE_CURVE ( 'NONE', #21459, #76682, #18235, .T. ) ;
#98089=DIRECTION ( 'NONE',  ( -0.000000000000000000, 1.000000000000000000, -0.000000000000000000 ) ) ;
#98448=ORIENTED_EDGE ( 'NONE', *, *, #29085, .T. ) ;
#98488=EDGE_CURVE ( 'NONE', #76546, #102801, #48855, .T. ) ;
#98499=DIRECTION ( 'NONE',  ( 0.8660254037844390407, 0.000000000000000000, -0.4999999999999991673 ) ) ;
#98862=EDGE_LOOP ( 'NONE', ( #129153, #25818, #92745, #13423 ) ) ;
#99000=CARTESIAN_POINT ( 'NONE',  ( 108.0000000000000142, 8.500000000000000000, -0.2500000000000000000 ) ) ;
#99052=MANIFOLD_SOLID_BREP ( 'Cut-Extrude-Thin1', #68669 ) ;
#99342=ORIENTED_EDGE ( 'NONE', *, *, #55661, .T. ) ;
#99774=CYLINDRICAL_SURFACE ( 'NONE', #35042, 2.249999999999996891 ) ;
#100184=ADVANCED_FACE ( 'NONE', ( #57403 ), #76401, .F. ) ;
#100196=SURFACE_STYLE_USAGE ( .BOTH. , #41929 ) ;
#100366=LINE ( 'NONE', #89887, #79859 ) ;
#100790=DIRECTION ( 'NONE',  ( -0.000000000000000000, -1.000000000000000000, -0.000000000000000000 ) ) ;
#100816=FILL_AREA_STYLE_COLOUR ( '', #41524 ) ;
#101005=CARTESIAN_POINT ( 'NONE',  ( 108.0000000000000142, 9.000000000000001776, 0.2500000000000000000 ) ) ;
#101076=DIRECTION ( 'NONE',  ( -0.000000000000000000, -1.000000000000000000, -0.000000000000000000 ) ) ;
#101209=DIRECTION ( 'NONE',  ( 0.000000000000000000, 0.000000000000000000, -1.000000000000000000 ) ) ;
#101383=CIRCLE ( 'NONE', #122319, 2.750000000000002665 ) ;
#101588=CYLINDRICAL_SURFACE ( 'NONE', #37329, 2.749999999999997335 ) ;
#101771=ADVANCED_FACE ( 'NONE', ( #61792 ), #110230, .F. ) ;
#102084=EDGE_CURVE ( 'NONE', #112645, #21459, #117159, .T. ) ;
#102127=( NAMED_UNIT ( * ) SI_UNIT ( $, .STERADIAN. ) SOLID_ANGLE_UNIT ( ) );
#102159=ORIENTED_EDGE ( 'NONE', *, *, #1377, .T. ) ;
#102249=LINE ( 'NONE', #91774, #38166 ) ;
#102627=EDGE_CURVE ( 'NONE', #108936, #107284, #88321, .T. ) ;
#102801=VERTEX_POINT ( 'NONE', #66612 ) ;
#102836=DIRECTION ( 'NONE',  ( 0.000000000000000000, 0.000000000000000000, 1.000000000000000000 ) ) ;
#102854=DIRECTION ( 'NONE',  ( -0.000000000000000000, 1.000000000000000000, -0.000000000000000000 ) ) ;
#102869=DIRECTION ( 'NONE',  ( -0.000000000000000000, 1.000000000000000000, -0.000000000000000000 ) ) ;
#102884=ADVANCED_FACE ( 'NONE', ( #97367 ), #65214, .T. ) ;
#103192=ORIENTED_EDGE ( 'NONE', *, *, #8522, .T. ) ;
#103329=FACE_OUTER_BOUND ( 'NONE', #78765, .T. ) ;
#103489=CARTESIAN_POINT ( 'NONE',  ( 106.0514428414850272, 8.500000000000000000, 1.125000000000000444 ) ) ;
#104499=ORIENTED_EDGE ( 'NONE', *, *, #69347, .F. ) ;
#104542=ADVANCED_FACE ( 'NONE', ( #87523 ), #37163, .T. ) ;
#104719=DIRECTION ( 'NONE',  ( -1.000000000000000000, 0.000000000000000000, 1.224646799147352221E-16 ) ) ;
#105671=VECTOR ( 'NONE', #114082, 1000.000000000000000 ) ;
#105856=CARTESIAN_POINT ( 'NONE',  ( 108.0000000000000142, 8.500000000000000000, 0.000000000000000000 ) ) ;
#106005=EDGE_CURVE ( 'NONE', #45696, #2267, #121505, .T. ) ;
#106077=AXIS2_PLACEMENT_3D ( 'NONE', #86120, #25272, #126061 ) ;
#106510=ORIENTED_EDGE ( 'NONE', *, *, #63862, .F. ) ;
#106834=EDGE_CURVE ( 'NONE', #50498, #112645, #23418, .T. ) ;
#106851=DIRECTION ( 'NONE',  ( -0.000000000000000000, -1.000000000000000000, -0.000000000000000000 ) ) ;
#106872=VERTEX_POINT ( 'NONE', #99000 ) ;
#106935=AXIS2_PLACEMENT_3D ( 'NONE', #31821, #61287, #101209 ) ;
#107284=VERTEX_POINT ( 'NONE', #45888 ) ;
#107654=ADVANCED_FACE ( 'NONE', ( #61934 ), #49540, .T. ) ;
#108296=AXIS2_PLACEMENT_3D ( 'NONE', #10644, #90516, #80718 ) ;
#108331=LINE ( 'NONE', #58606, #123902 ) ;
#108539=VECTOR ( 'NONE', #58552, 1000.000000000000227 ) ;
#108567=PRODUCT_CONTEXT ( 'NONE', #2834, 'mechanical' ) ;
#108597=ADVANCED_BREP_SHAPE_REPRESENTATION ( '', ( #99052, #108296 ), #5971 ) ;
#108737=ORIENTED_EDGE ( 'NONE', *, *, #8522, .F. ) ;
#108787=CARTESIAN_POINT ( 'NONE',  ( 108.0000000000000142, 9.000000000000001776, 0.000000000000000000 ) ) ;
#108936=VERTEX_POINT ( 'NONE', #18780 ) ;
#108996=ORIENTED_EDGE ( 'NONE', *, *, #77893, .T. ) ;
#109201=CARTESIAN_POINT ( 'NONE',  ( 108.0000000000000142, 5.000000000000000000, 5.000000000000004441 ) ) ;
#109269=LINE ( 'NONE', #127625, #63036 ) ;
#109687=VERTEX_POINT ( 'NONE', #95118 ) ;
#109932=CARTESIAN_POINT ( 'NONE',  ( 105.0000000000000142, 9.000000000000001776, 0.2500000000000003886 ) ) ;
#110230=PLANE ( 'NONE',  #87835 ) ;
#110231=DIRECTION ( 'NONE',  ( -0.000000000000000000, 1.000000000000000000, -0.000000000000000000 ) ) ;
#110535=EDGE_LOOP ( 'NONE', ( #11396, #3340, #40340, #15253 ) ) ;
#110733=CIRCLE ( 'NONE', #77288, 5.000000000000004441 ) ;
#111518=VECTOR ( 'NONE', #76356, 1000.000000000000000 ) ;
#111695=LINE ( 'NONE', #3667, #96471 ) ;
#112095=DIRECTION ( 'NONE',  ( 1.000000000000000000, 0.000000000000000000, -1.776356839400246520E-15 ) ) ;
#112645=VERTEX_POINT ( 'NONE', #117778 ) ;
#112859=CIRCLE ( 'NONE', #81557, 0.5000000000000004441 ) ;
#113114=CARTESIAN_POINT ( 'NONE',  ( 108.0000000000000142, 8.500000000000000000, 0.000000000000000000 ) ) ;
#113227=EDGE_CURVE ( 'NONE', #115931, #109687, #93979, .T. ) ;
#113422=EDGE_CURVE ( 'NONE', #45696, #21874, #112859, .T. ) ;
#113484=ORIENTED_EDGE ( 'NONE', *, *, #51210, .F. ) ;
#113671=ADVANCED_FACE ( 'NONE', ( #128308 ), #77886, .T. ) ;
#113715=CARTESIAN_POINT ( 'NONE',  ( 105.6184301395928031, 9.000000000000001776, 1.375000000000001110 ) ) ;
#113814=FACE_OUTER_BOUND ( 'NONE', #74625, .T. ) ;
#113939=CARTESIAN_POINT ( 'NONE',  ( 106.0514428414850272, 9.000000000000001776, -1.125000000000000222 ) ) ;
#114082=DIRECTION ( 'NONE',  ( -0.000000000000000000, 1.000000000000000000, -0.000000000000000000 ) ) ;
#114103=CARTESIAN_POINT ( 'NONE',  ( 108.0000000000000142, 8.500000000000000000, -2.749999999999997335 ) ) ;
#114243=EDGE_CURVE ( 'NONE', #121831, #2267, #71472, .T. ) ;
#114645=MECHANICAL_DESIGN_GEOMETRIC_PRESENTATION_REPRESENTATION('',(#33199),#74948);
#114837=CARTESIAN_POINT ( 'NONE',  ( 108.0000000000000142, 9.000000000000001776, -2.249999999999996891 ) ) ;
#115118=CARTESIAN_POINT ( 'NONE',  ( 108.0000000000000142, 8.500000000000000000, -0.2500000000000000000 ) ) ;
#115553=ORIENTED_EDGE ( 'NONE', *, *, #102627, .T. ) ;
#115931=VERTEX_POINT ( 'NONE', #114837 ) ;
#116544=( GEOMETRIC_REPRESENTATION_CONTEXT ( 3 ) GLOBAL_UNCERTAINTY_ASSIGNED_CONTEXT ( ( #6047 ) ) GLOBAL_UNIT_ASSIGNED_CONTEXT ( ( #11976, #70266, #1508 ) ) REPRESENTATION_CONTEXT ( 'NONE', 'WORKASPACE' ) );
#116619=VECTOR ( 'NONE', #73521, 1000.000000000000000 ) ;
#116796=VECTOR ( 'NONE', #19205, 1000.000000000000000 ) ;
#116854=DIRECTION ( 'NONE',  ( -0.000000000000000000, -1.000000000000000000, -0.000000000000000000 ) ) ;
#116969=EDGE_LOOP ( 'NONE', ( #74810, #102159, #83889, #104499 ) ) ;
#117159=CIRCLE ( 'NONE', #60761, 2.750000000000002665 ) ;
#117219=EDGE_CURVE ( 'NONE', #121539, #108936, #66412, .T. ) ;
#117421=LINE ( 'NONE', #16016, #22796 ) ;
#117555=CARTESIAN_POINT ( 'NONE',  ( 108.0000000000000142, 9.000000000000001776, 0.000000000000000000 ) ) ;
#117778=CARTESIAN_POINT ( 'NONE',  ( 108.0000000000000142, 8.500000000000000000, -2.749999999999997335 ) ) ;
#117792=EDGE_CURVE ( 'NONE', #41830, #107284, #63700, .T. ) ;
#117804=DIRECTION ( 'NONE',  ( -0.000000000000000000, 1.000000000000000000, 0.000000000000000000 ) ) ;
#118389=ORIENTED_EDGE ( 'NONE', *, *, #77893, .F. ) ;
#118797=LINE ( 'NONE', #119430, #51191 ) ;
#118857=ADVANCED_FACE ( 'NONE', ( #59873 ), #99774, .T. ) ;
#119036=SHAPE_DEFINITION_REPRESENTATION ( #97200, #89551 ) ;
#119430=CARTESIAN_POINT ( 'NONE',  ( 108.0000000000000142, 8.500000000000000000, -0.2500000000000000000 ) ) ;
#120319=DIRECTION ( 'NONE',  ( 0.000000000000000000, 0.000000000000000000, 1.000000000000000000 ) ) ;
#120477=SURFACE_STYLE_FILL_AREA ( #91657 ) ;
#120558=CARTESIAN_POINT ( 'NONE',  ( 108.0000000000000142, 8.500000000000000000, 4.500000000000003553 ) ) ;
#120684=CARTESIAN_POINT ( 'NONE',  ( 106.0514428414850272, 8.500000000000000000, -1.125000000000000222 ) ) ;
#120884=VECTOR ( 'NONE', #24135, 1000.000000000000000 ) ;
#121290=EDGE_LOOP ( 'NONE', ( #46623, #3313, #10960, #52694 ) ) ;
#121505=LINE ( 'NONE', #12204, #21087 ) ;
#121536=VERTEX_POINT ( 'NONE', #31472 ) ;
#121539=VERTEX_POINT ( 'NONE', #51125 ) ;
#121561=VECTOR ( 'NONE', #68700, 1000.000000000000000 ) ;
#121739=ORIENTED_EDGE ( 'NONE', *, *, #51210, .T. ) ;
#121831=VERTEX_POINT ( 'NONE', #86349 ) ;
#121989=AXIS2_PLACEMENT_3D ( 'NONE', #51679, #13659, #122354 ) ;
#122223=AXIS2_PLACEMENT_3D ( 'NONE', #66818, #94356, #34828 ) ;
#122319=AXIS2_PLACEMENT_3D ( 'NONE', #117555, #881, #27919 ) ;
#122354=DIRECTION ( 'NONE',  ( -0.8660254037844391517, 0.000000000000000000, -0.4999999999999992228 ) ) ;
#122837=ORIENTED_EDGE ( 'NONE', *, *, #69347, .T. ) ;
#123182=ORIENTED_EDGE ( 'NONE', *, *, #50333, .F. ) ;
#123568=DIRECTION ( 'NONE',  ( 0.000000000000000000, 0.000000000000000000, 1.000000000000000000 ) ) ;
#123902=VECTOR ( 'NONE', #98499, 1000.000000000000227 ) ;
#124091=ORIENTED_EDGE ( 'NONE', *, *, #113227, .F. ) ;
#124151=CARTESIAN_POINT ( 'NONE',  ( 105.6184301395928031, 8.500000000000000000, 1.375000000000001110 ) ) ;
#124257=PLANE ( 'NONE',  #55852 ) ;
#124816=AXIS2_PLACEMENT_3D ( 'NONE', #81663, #11637, #19520 ) ;
#126061=DIRECTION ( 'NONE',  ( 1.000000000000000000, 0.000000000000000000, 0.000000000000000000 ) ) ;
#126359=CARTESIAN_POINT ( 'NONE',  ( 108.0000000000000142, 8.500000000000000000, 0.000000000000000000 ) ) ;
#126416=CIRCLE ( 'NONE', #68004, 2.250000000000001776 ) ;
#126596=ADVANCED_FACE ( 'NONE', ( #5975 ), #95666, .T. ) ;
#126781=VECTOR ( 'NONE', #64110, 1000.000000000000000 ) ;
#126869=DIRECTION ( 'NONE',  ( 0.000000000000000000, 1.000000000000000000, 0.000000000000000000 ) ) ;
#127046=CIRCLE ( 'NONE', #93589, 2.250000000000001776 ) ;
#127262=DIRECTION ( 'NONE',  ( -1.224646799147352221E-16, 0.000000000000000000, -1.000000000000000000 ) ) ;
#127274=ORIENTED_EDGE ( 'NONE', *, *, #89462, .F. ) ;
#127625=CARTESIAN_POINT ( 'NONE',  ( 105.6184301395928031, 8.500000000000000000, 1.375000000000001110 ) ) ;
#127871=CARTESIAN_POINT ( 'NONE',  ( 108.0000000000000142, 8.500000000000000000, 0.000000000000000000 ) ) ;
#127982=AXIS2_PLACEMENT_3D ( 'NONE', #76021, #56374, #46549 ) ;
#128177=ORIENTED_EDGE ( 'NONE', *, *, #65966, .T. ) ;
#128308=FACE_OUTER_BOUND ( 'NONE', #24976, .T. ) ;
#128617=ORIENTED_EDGE ( 'NONE', *, *, #71108, .T. ) ;
#129153=ORIENTED_EDGE ( 'NONE', *, *, #86447, .F. ) ;
ENDSEC;
END-ISO-10303-21;
